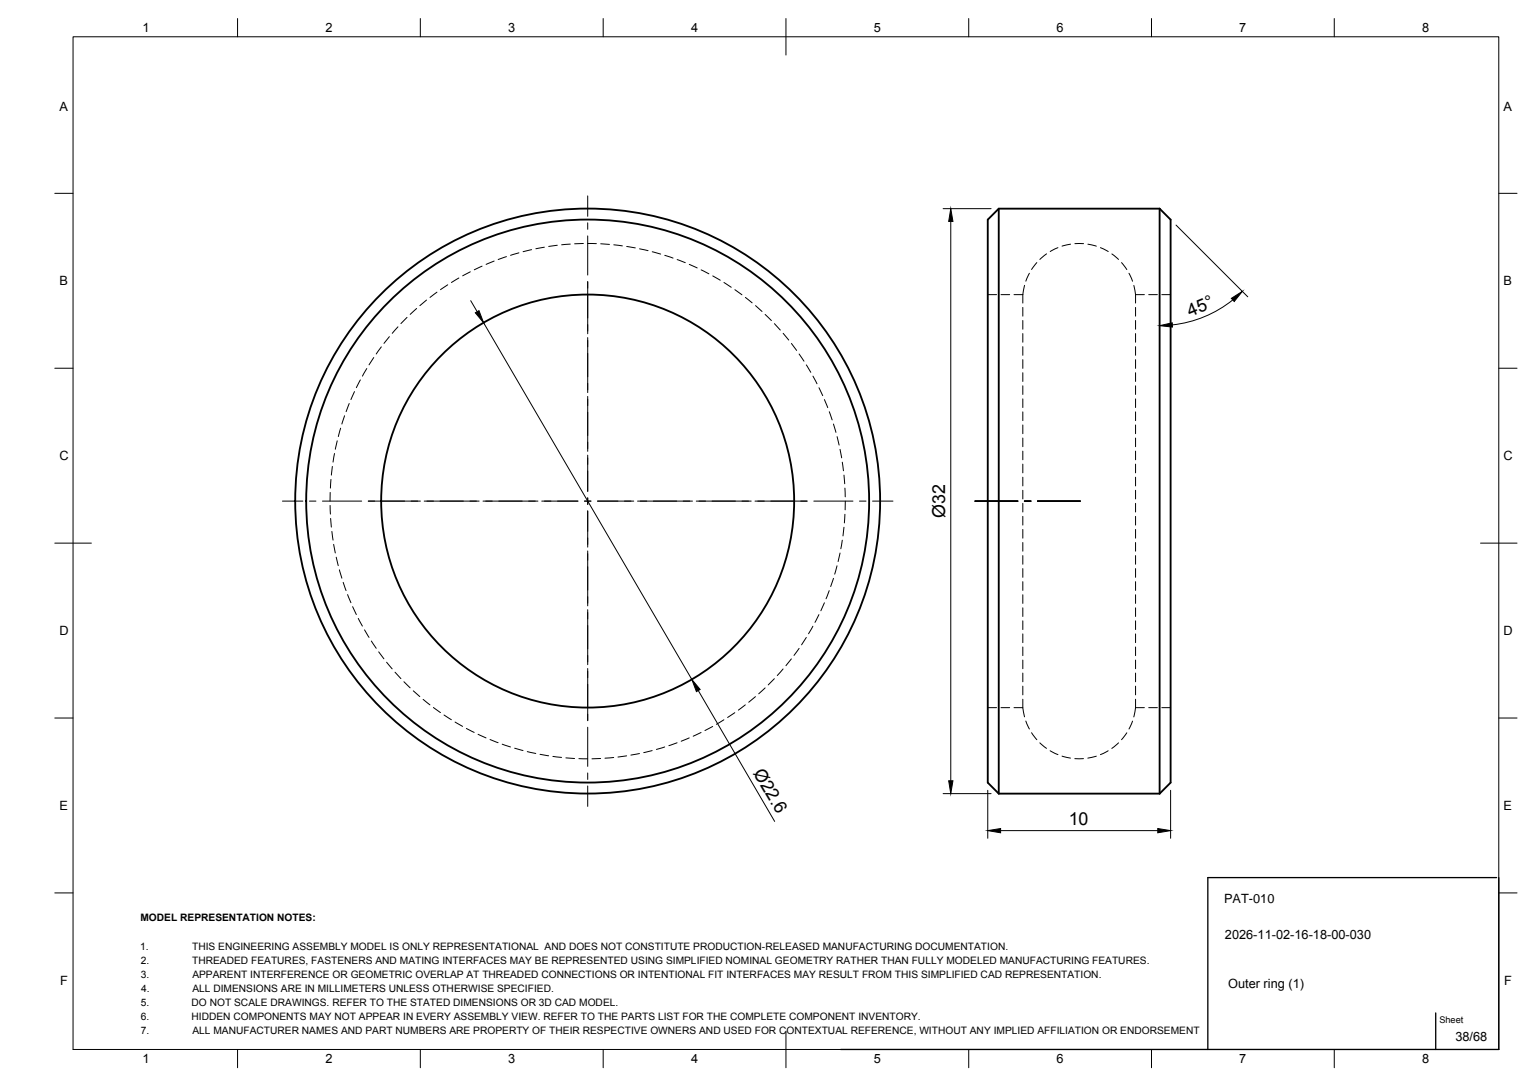
ISO-10303-21;
HEADER;
/* Generated by software containing ST-Developer
 * from STEP Tools, Inc. (www.steptools.com) 
 */

FILE_DESCRIPTION(
/* description */ ('Belt conveyor head drive unit'),
/* implementation_level */ '2;1');

FILE_NAME(
/* name */ 'Outer ring (1).step',
/* time_stamp */ '2026-10-28T03:26:19-07:00',
/* author */ (''),
/* organization */ (''),
/* preprocessor_version */ 'ST-DEVELOPER v20.2',
/* originating_system */ 'Autodesk Translation Framework v15.17.0.0',
/* authorisation */ '');

FILE_SCHEMA (('AUTOMOTIVE_DESIGN { 1 0 10303 214 3 1 1 }'));
ENDSEC;

DATA;
#10=MECHANICAL_DESIGN_GEOMETRIC_PRESENTATION_REPRESENTATION('',(#889),#27069);
#687=CONICAL_SURFACE('',#15386,1.57,0.785398163397449);
#688=CONICAL_SURFACE('',#15390,1.57,0.785398163397449);
#708=TOROIDAL_SURFACE('',#15375,1.1,0.309556);
#743=SHAPE_REPRESENTATION_RELATIONSHIP('SRR','None',#27389,#812);
#812=ADVANCED_BREP_SHAPE_REPRESENTATION('',(#973),#27031);
#889=STYLED_ITEM('',(#27797),#973);
#973=MANIFOLD_SOLID_BREP('Body1',#13755);
#1164=FACE_BOUND('',#2968,.T.);
#1165=FACE_BOUND('',#2973,.T.);
#1468=PLANE('',#15383);
#1469=PLANE('',#15392);
#2013=FACE_OUTER_BOUND('',#2965,.T.);
#2014=FACE_OUTER_BOUND('',#2966,.T.);
#2015=FACE_OUTER_BOUND('',#2967,.T.);
#2016=FACE_OUTER_BOUND('',#2969,.T.);
#2017=FACE_OUTER_BOUND('',#2970,.T.);
#2018=FACE_OUTER_BOUND('',#2971,.T.);
#2019=FACE_OUTER_BOUND('',#2972,.T.);
#2020=FACE_OUTER_BOUND('',#2974,.T.);
#2965=EDGE_LOOP('',(#10586,#10587,#10588,#10589,#10590,#10591));
#2966=EDGE_LOOP('',(#10592,#10593,#10594,#10595,#10596));
#2967=EDGE_LOOP('',(#10597));
#2968=EDGE_LOOP('',(#10598));
#2969=EDGE_LOOP('',(#10599,#10600,#10601,#10602));
#2970=EDGE_LOOP('',(#10603,#10604,#10605,#10606));
#2971=EDGE_LOOP('',(#10607,#10608,#10609,#10610));
#2972=EDGE_LOOP('',(#10611));
#2973=EDGE_LOOP('',(#10612));
#2974=EDGE_LOOP('',(#10613,#10614,#10615,#10616,#10617));
#3905=LINE('',#23109,#4697);
#3906=LINE('',#23118,#4698);
#3907=LINE('',#23122,#4699);
#3908=LINE('',#23126,#4700);
#3909=LINE('',#23129,#4701);
#4697=VECTOR('',#18483,1.129765);
#4698=VECTOR('',#18494,1.57);
#4699=VECTOR('',#18499,1.6);
#4700=VECTOR('',#18504,1.57);
#4701=VECTOR('',#18509,1.129765);
#5471=CIRCLE('',#15376,1.129765);
#5472=CIRCLE('',#15377,1.129765);
#5473=CIRCLE('',#15378,0.309556);
#5474=CIRCLE('',#15379,1.129765);
#5475=CIRCLE('',#15380,1.129765);
#5476=CIRCLE('',#15382,1.129765);
#5477=CIRCLE('',#15384,1.54);
#5478=CIRCLE('',#15385,1.129765);
#5479=CIRCLE('',#15387,1.6);
#5480=CIRCLE('',#15389,1.6);
#5481=CIRCLE('',#15391,1.54);
#6503=VERTEX_POINT('',#23097);
#6504=VERTEX_POINT('',#23098);
#6505=VERTEX_POINT('',#23101);
#6506=VERTEX_POINT('',#23103);
#6507=VERTEX_POINT('',#23107);
#6508=VERTEX_POINT('',#23111);
#6509=VERTEX_POINT('',#23113);
#6510=VERTEX_POINT('',#23116);
#6511=VERTEX_POINT('',#23120);
#6512=VERTEX_POINT('',#23124);
#7985=EDGE_CURVE('',#6503,#6504,#5471,.T.);
#7986=EDGE_CURVE('',#6504,#6503,#5472,.T.);
#7987=EDGE_CURVE('',#6504,#6505,#5473,.T.);
#7988=EDGE_CURVE('',#6506,#6505,#5474,.T.);
#7989=EDGE_CURVE('',#6505,#6506,#5475,.T.);
#7990=EDGE_CURVE('',#6507,#6507,#5476,.T.);
#7991=EDGE_CURVE('',#6507,#6506,#3905,.T.);
#7992=EDGE_CURVE('',#6508,#6508,#5477,.T.);
#7993=EDGE_CURVE('',#6509,#6509,#5478,.T.);
#7994=EDGE_CURVE('',#6510,#6510,#5479,.T.);
#7995=EDGE_CURVE('',#6510,#6508,#3906,.T.);
#7996=EDGE_CURVE('',#6511,#6511,#5480,.T.);
#7997=EDGE_CURVE('',#6511,#6510,#3907,.T.);
#7998=EDGE_CURVE('',#6512,#6512,#5481,.T.);
#7999=EDGE_CURVE('',#6512,#6511,#3908,.T.);
#8000=EDGE_CURVE('',#6503,#6509,#3909,.T.);
#10586=ORIENTED_EDGE('',*,*,#7985,.F.);
#10587=ORIENTED_EDGE('',*,*,#7986,.F.);
#10588=ORIENTED_EDGE('',*,*,#7987,.T.);
#10589=ORIENTED_EDGE('',*,*,#7988,.F.);
#10590=ORIENTED_EDGE('',*,*,#7989,.F.);
#10591=ORIENTED_EDGE('',*,*,#7987,.F.);
#10592=ORIENTED_EDGE('',*,*,#7990,.T.);
#10593=ORIENTED_EDGE('',*,*,#7991,.T.);
#10594=ORIENTED_EDGE('',*,*,#7988,.T.);
#10595=ORIENTED_EDGE('',*,*,#7989,.T.);
#10596=ORIENTED_EDGE('',*,*,#7991,.F.);
#10597=ORIENTED_EDGE('',*,*,#7992,.F.);
#10598=ORIENTED_EDGE('',*,*,#7993,.T.);
#10599=ORIENTED_EDGE('',*,*,#7994,.F.);
#10600=ORIENTED_EDGE('',*,*,#7995,.T.);
#10601=ORIENTED_EDGE('',*,*,#7992,.T.);
#10602=ORIENTED_EDGE('',*,*,#7995,.F.);
#10603=ORIENTED_EDGE('',*,*,#7996,.F.);
#10604=ORIENTED_EDGE('',*,*,#7997,.T.);
#10605=ORIENTED_EDGE('',*,*,#7994,.T.);
#10606=ORIENTED_EDGE('',*,*,#7997,.F.);
#10607=ORIENTED_EDGE('',*,*,#7998,.F.);
#10608=ORIENTED_EDGE('',*,*,#7999,.T.);
#10609=ORIENTED_EDGE('',*,*,#7996,.T.);
#10610=ORIENTED_EDGE('',*,*,#7999,.F.);
#10611=ORIENTED_EDGE('',*,*,#7998,.T.);
#10612=ORIENTED_EDGE('',*,*,#7990,.F.);
#10613=ORIENTED_EDGE('',*,*,#7985,.T.);
#10614=ORIENTED_EDGE('',*,*,#7986,.T.);
#10615=ORIENTED_EDGE('',*,*,#8000,.T.);
#10616=ORIENTED_EDGE('',*,*,#7993,.F.);
#10617=ORIENTED_EDGE('',*,*,#8000,.F.);
#12692=CYLINDRICAL_SURFACE('',#15381,1.129765);
#12693=CYLINDRICAL_SURFACE('',#15388,1.6);
#12694=CYLINDRICAL_SURFACE('',#15393,1.129765);
#13292=ADVANCED_FACE('',(#2013),#708,.F.);
#13293=ADVANCED_FACE('',(#2014),#12692,.F.);
#13294=ADVANCED_FACE('',(#2015,#1164),#1468,.T.);
#13295=ADVANCED_FACE('',(#2016),#687,.T.);
#13296=ADVANCED_FACE('',(#2017),#12693,.T.);
#13297=ADVANCED_FACE('',(#2018),#688,.T.);
#13298=ADVANCED_FACE('',(#2019,#1165),#1469,.T.);
#13299=ADVANCED_FACE('',(#2020),#12694,.F.);
#13755=CLOSED_SHELL('',(#13292,#13293,#13294,#13295,#13296,#13297,#13298,
#13299));
#15374=AXIS2_PLACEMENT_3D('',#23095,#18465,#18466);
#15375=AXIS2_PLACEMENT_3D('',#23096,#18467,#18468);
#15376=AXIS2_PLACEMENT_3D('',#23099,#18469,#18470);
#15377=AXIS2_PLACEMENT_3D('',#23100,#18471,#18472);
#15378=AXIS2_PLACEMENT_3D('',#23102,#18473,#18474);
#15379=AXIS2_PLACEMENT_3D('',#23104,#18475,#18476);
#15380=AXIS2_PLACEMENT_3D('',#23105,#18477,#18478);
#15381=AXIS2_PLACEMENT_3D('',#23106,#18479,#18480);
#15382=AXIS2_PLACEMENT_3D('',#23108,#18481,#18482);
#15383=AXIS2_PLACEMENT_3D('',#23110,#18484,#18485);
#15384=AXIS2_PLACEMENT_3D('',#23112,#18486,#18487);
#15385=AXIS2_PLACEMENT_3D('',#23114,#18488,#18489);
#15386=AXIS2_PLACEMENT_3D('',#23115,#18490,#18491);
#15387=AXIS2_PLACEMENT_3D('',#23117,#18492,#18493);
#15388=AXIS2_PLACEMENT_3D('',#23119,#18495,#18496);
#15389=AXIS2_PLACEMENT_3D('',#23121,#18497,#18498);
#15390=AXIS2_PLACEMENT_3D('',#23123,#18500,#18501);
#15391=AXIS2_PLACEMENT_3D('',#23125,#18502,#18503);
#15392=AXIS2_PLACEMENT_3D('',#23127,#18505,#18506);
#15393=AXIS2_PLACEMENT_3D('',#23128,#18507,#18508);
#18465=DIRECTION('axis',(0.,0.,1.));
#18466=DIRECTION('refdir',(1.,0.,0.));
#18467=DIRECTION('center_axis',(0.,-1.,0.));
#18468=DIRECTION('ref_axis',(0.,0.,-1.));
#18469=DIRECTION('center_axis',(0.,-1.,0.));
#18470=DIRECTION('ref_axis',(1.,0.,0.));
#18471=DIRECTION('center_axis',(0.,-1.,0.));
#18472=DIRECTION('ref_axis',(1.,0.,0.));
#18473=DIRECTION('center_axis',(1.,0.,1.22464679914735E-16));
#18474=DIRECTION('ref_axis',(-1.22464679914735E-16,0.,1.));
#18475=DIRECTION('center_axis',(0.,1.,0.));
#18476=DIRECTION('ref_axis',(1.,0.,0.));
#18477=DIRECTION('center_axis',(0.,1.,0.));
#18478=DIRECTION('ref_axis',(1.,0.,0.));
#18479=DIRECTION('center_axis',(0.,-1.,0.));
#18480=DIRECTION('ref_axis',(1.,0.,0.));
#18481=DIRECTION('center_axis',(0.,-1.,0.));
#18482=DIRECTION('ref_axis',(1.,0.,0.));
#18483=DIRECTION('',(0.,1.,0.));
#18484=DIRECTION('center_axis',(0.,1.,0.));
#18485=DIRECTION('ref_axis',(0.,0.,1.));
#18486=DIRECTION('center_axis',(0.,-1.,0.));
#18487=DIRECTION('ref_axis',(1.,0.,0.));
#18488=DIRECTION('center_axis',(0.,-1.,0.));
#18489=DIRECTION('ref_axis',(1.,0.,0.));
#18490=DIRECTION('center_axis',(0.,-1.,0.));
#18491=DIRECTION('ref_axis',(1.,0.,0.));
#18492=DIRECTION('center_axis',(0.,-1.,0.));
#18493=DIRECTION('ref_axis',(1.,0.,0.));
#18494=DIRECTION('',(0.707106781186548,0.707106781186547,8.65956056235494E-17));
#18495=DIRECTION('center_axis',(0.,-1.,0.));
#18496=DIRECTION('ref_axis',(1.,0.,0.));
#18497=DIRECTION('center_axis',(0.,-1.,0.));
#18498=DIRECTION('ref_axis',(1.,0.,0.));
#18499=DIRECTION('',(0.,1.,0.));
#18500=DIRECTION('center_axis',(0.,1.,0.));
#18501=DIRECTION('ref_axis',(1.,0.,0.));
#18502=DIRECTION('center_axis',(0.,-1.,0.));
#18503=DIRECTION('ref_axis',(1.,0.,0.));
#18504=DIRECTION('',(-0.707106781186548,0.707106781186547,-8.65956056235494E-17));
#18505=DIRECTION('center_axis',(0.,-1.,0.));
#18506=DIRECTION('ref_axis',(0.,0.,-1.));
#18507=DIRECTION('center_axis',(0.,-1.,0.));
#18508=DIRECTION('ref_axis',(1.,0.,0.));
#18509=DIRECTION('',(0.,1.,0.));
#23095=CARTESIAN_POINT('',(0.,0.,0.));
#23096=CARTESIAN_POINT('Origin',(0.,0.,0.));
#23097=CARTESIAN_POINT('',(-1.129765,0.308121667383195,-1.38356309103871E-16));
#23098=CARTESIAN_POINT('',(-1.38356309103871E-16,0.308121667383195,1.129765));
#23099=CARTESIAN_POINT('Origin',(0.,0.308121667383195,0.));
#23100=CARTESIAN_POINT('Origin',(0.,0.308121667383195,0.));
#23101=CARTESIAN_POINT('',(-1.38356309103871E-16,-0.308121667383195,1.129765));
#23102=CARTESIAN_POINT('Origin',(-1.34711147906209E-16,0.,1.1));
#23103=CARTESIAN_POINT('',(-1.129765,-0.308121667383195,1.38356309103871E-16));
#23104=CARTESIAN_POINT('Origin',(0.,-0.308121667383195,0.));
#23105=CARTESIAN_POINT('Origin',(0.,-0.308121667383195,0.));
#23106=CARTESIAN_POINT('Origin',(0.,0.,0.));
#23107=CARTESIAN_POINT('',(-1.129765,-0.5,-1.38356309103871E-16));
#23108=CARTESIAN_POINT('Origin',(0.,-0.5,0.));
#23109=CARTESIAN_POINT('',(-1.129765,0.,-1.38356309103871E-16));
#23110=CARTESIAN_POINT('Origin',(1.54,0.5,0.));
#23111=CARTESIAN_POINT('',(-1.54,0.5,-1.88595607068692E-16));
#23112=CARTESIAN_POINT('Origin',(0.,0.5,0.));
#23113=CARTESIAN_POINT('',(-1.129765,0.5,-1.38356309103871E-16));
#23114=CARTESIAN_POINT('Origin',(0.,0.5,0.));
#23115=CARTESIAN_POINT('Origin',(0.,0.47,0.));
#23116=CARTESIAN_POINT('',(-1.6,0.44,-1.95943487863577E-16));
#23117=CARTESIAN_POINT('Origin',(0.,0.44,0.));
#23118=CARTESIAN_POINT('',(-1.57,0.47,-1.92269547466134E-16));
#23119=CARTESIAN_POINT('Origin',(0.,0.,0.));
#23120=CARTESIAN_POINT('',(-1.6,-0.44,-1.95943487863577E-16));
#23121=CARTESIAN_POINT('Origin',(0.,-0.44,0.));
#23122=CARTESIAN_POINT('',(-1.6,0.,-1.95943487863577E-16));
#23123=CARTESIAN_POINT('Origin',(0.,-0.47,0.));
#23124=CARTESIAN_POINT('',(-1.54,-0.5,-1.88595607068692E-16));
#23125=CARTESIAN_POINT('Origin',(0.,-0.5,0.));
#23126=CARTESIAN_POINT('',(-1.57,-0.47,-1.92269547466134E-16));
#23127=CARTESIAN_POINT('Origin',(1.129765,-0.5,0.));
#23128=CARTESIAN_POINT('Origin',(0.,0.,0.));
#23129=CARTESIAN_POINT('',(-1.129765,0.,-1.38356309103871E-16));
#26954=UNCERTAINTY_MEASURE_WITH_UNIT(LENGTH_MEASURE(0.001),#27070,
'DISTANCE_ACCURACY_VALUE',
'Maximum model space distance between geometric entities at asserted c
onnectivities');
#26992=UNCERTAINTY_MEASURE_WITH_UNIT(LENGTH_MEASURE(0.001),#27070,
'DISTANCE_ACCURACY_VALUE',
'Maximum model space distance between geometric entities at asserted c
onnectivities');
#27031=(
GEOMETRIC_REPRESENTATION_CONTEXT(3)
GLOBAL_UNCERTAINTY_ASSIGNED_CONTEXT((#26954))
GLOBAL_UNIT_ASSIGNED_CONTEXT((#27070,#27072,#27073))
REPRESENTATION_CONTEXT('','3D')
);
#27069=(
GEOMETRIC_REPRESENTATION_CONTEXT(3)
GLOBAL_UNCERTAINTY_ASSIGNED_CONTEXT((#26992))
GLOBAL_UNIT_ASSIGNED_CONTEXT((#27070,#27072,#27073))
REPRESENTATION_CONTEXT('','3D')
);
#27070=(
LENGTH_UNIT()
NAMED_UNIT(*)
SI_UNIT(.CENTI.,.METRE.)
);
#27072=(
NAMED_UNIT(*)
PLANE_ANGLE_UNIT()
SI_UNIT($,.RADIAN.)
);
#27073=(
NAMED_UNIT(*)
SI_UNIT($,.STERADIAN.)
SOLID_ANGLE_UNIT()
);
#27112=SHAPE_DEFINITION_REPRESENTATION(#27193,#27389);
#27193=PRODUCT_DEFINITION_SHAPE('',$,#27466);
#27389=SHAPE_REPRESENTATION('',(#15374),#27031);
#27427=PRODUCT_DEFINITION_CONTEXT('part definition',#27657,'design');
#27466=PRODUCT_DEFINITION('Outer ring (1)','Outer ring (1)',#27542,#27427);
#27542=PRODUCT_DEFINITION_FORMATION('',$,#27697);
#27657=APPLICATION_CONTEXT(
'Core Data for Automotive Mechanical Design Process');
#27658=PRODUCT_CONTEXT('part definition',#27657,'mechanical');
#27697=PRODUCT('Outer ring (1)','Outer ring (1)','Outer ring (1)',(#27658));
#27791=COLOUR_RGB('Grey',0.48,0.52,0.57);
#27792=FILL_AREA_STYLE_COLOUR('',#27791);
#27793=FILL_AREA_STYLE('',(#27792));
#27794=SURFACE_STYLE_FILL_AREA(#27793);
#27795=SURFACE_SIDE_STYLE('',(#27794));
#27796=SURFACE_STYLE_USAGE(.BOTH.,#27795);
#27797=PRESENTATION_STYLE_ASSIGNMENT((#27796));
ENDSEC;
END-ISO-10303-21;
